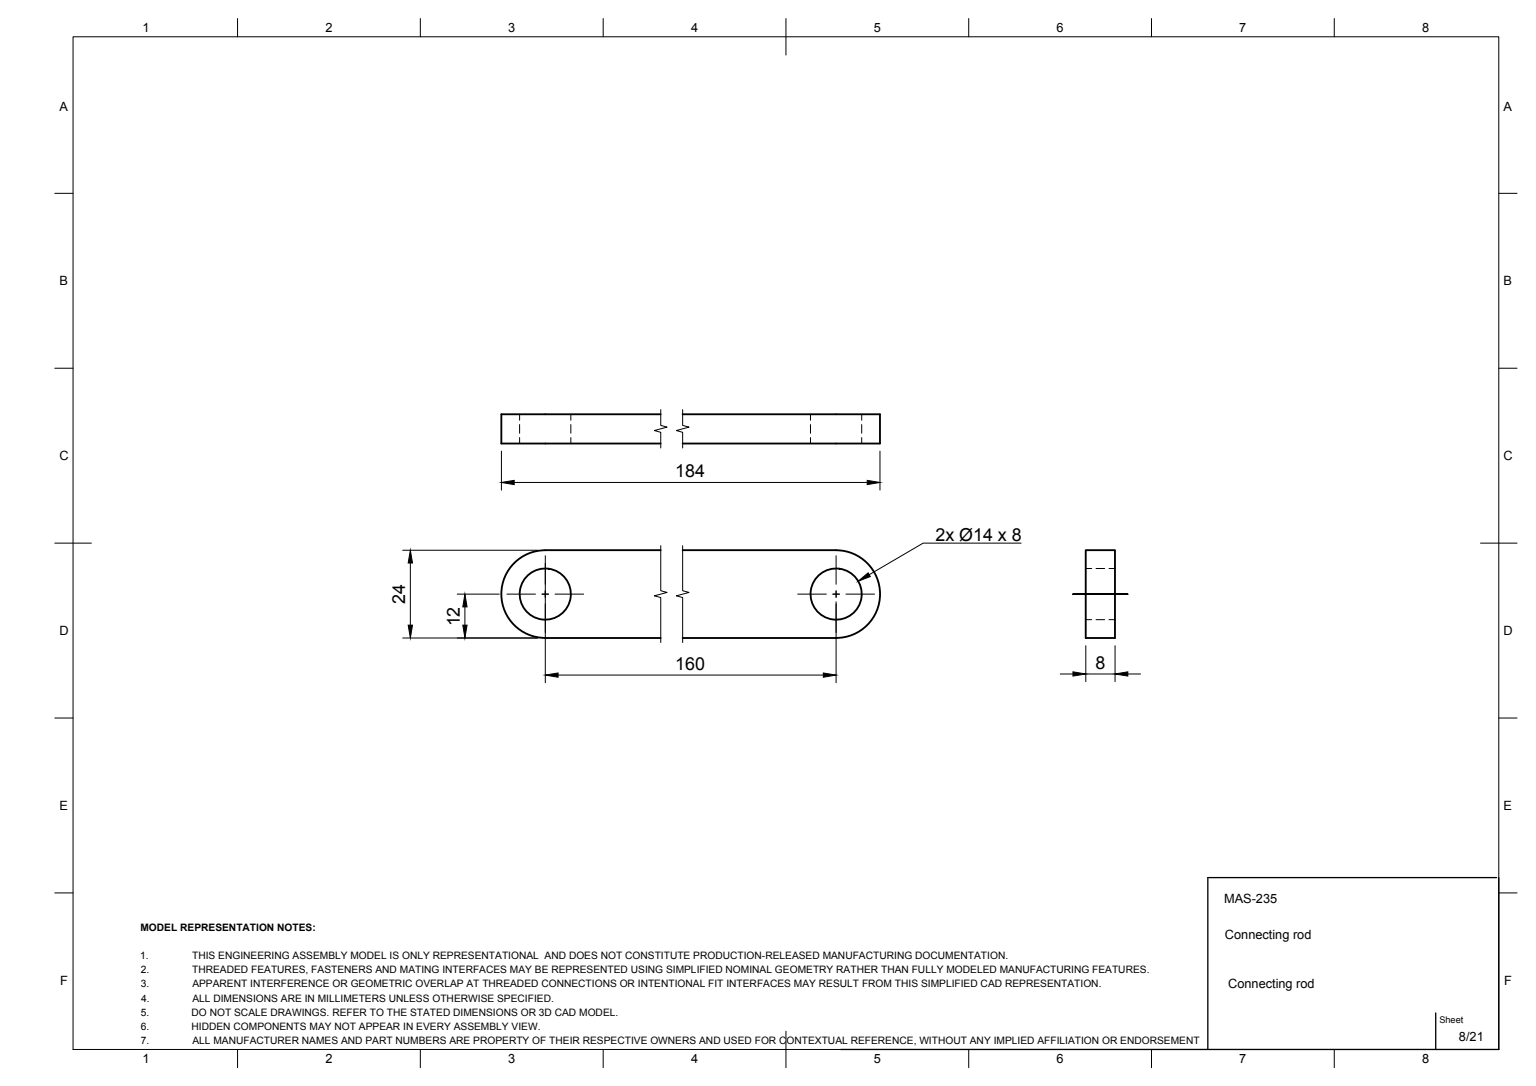
ISO-10303-21;
HEADER;
/* Generated by software containing ST-Developer
 * from STEP Tools, Inc. (www.steptools.com) 
 */

FILE_DESCRIPTION(
/* description */ ('Independent Whitworth quick-return mechanism. Crank radius40, ground-
center spacing80, lever180, connecting rod160, output guide X200. Nomi
nal stroke180 and long/short phase ratio2. Retained guide rods, replac
eable bearing sleeves and captured sliding shoe. No load or production
 rating assigned.'),
/* implementation_level */ '2;1');

FILE_NAME(
/* name */ 'Connecting rod.step',
/* time_stamp */ '2026-11-09T18:22:56-08:00',
/* author */ (''),
/* organization */ (''),
/* preprocessor_version */ 'ST-DEVELOPER v20.2',
/* originating_system */ 'Autodesk Translation Framework v15.17.0.0',
/* authorisation */ '');

FILE_SCHEMA (('AUTOMOTIVE_DESIGN { 1 0 10303 214 3 1 1 }'));
ENDSEC;

DATA;
#10=MECHANICAL_DESIGN_GEOMETRIC_PRESENTATION_REPRESENTATION('',(#224),#4388);
#184=SHAPE_REPRESENTATION_RELATIONSHIP('SRR','None',#4483,#204);
#204=ADVANCED_BREP_SHAPE_REPRESENTATION('',(#244),#4373);
#224=STYLED_ITEM('',(#4591),#244);
#244=MANIFOLD_SOLID_BREP('Body1',#2329);
#277=FACE_BOUND('',#613,.T.);
#278=FACE_BOUND('',#614,.T.);
#279=FACE_BOUND('',#616,.T.);
#280=FACE_BOUND('',#617,.T.);
#339=PLANE('',#2646);
#340=PLANE('',#2650);
#341=PLANE('',#2654);
#342=PLANE('',#2655);
#441=FACE_OUTER_BOUND('',#606,.T.);
#442=FACE_OUTER_BOUND('',#607,.T.);
#443=FACE_OUTER_BOUND('',#608,.T.);
#444=FACE_OUTER_BOUND('',#609,.T.);
#445=FACE_OUTER_BOUND('',#610,.T.);
#446=FACE_OUTER_BOUND('',#611,.T.);
#447=FACE_OUTER_BOUND('',#612,.T.);
#448=FACE_OUTER_BOUND('',#615,.T.);
#606=EDGE_LOOP('',(#1750,#1751,#1752,#1753));
#607=EDGE_LOOP('',(#1754,#1755,#1756,#1757));
#608=EDGE_LOOP('',(#1758,#1759,#1760,#1761));
#609=EDGE_LOOP('',(#1762,#1763,#1764,#1765));
#610=EDGE_LOOP('',(#1766,#1767,#1768,#1769));
#611=EDGE_LOOP('',(#1770,#1771,#1772,#1773));
#612=EDGE_LOOP('',(#1774,#1775,#1776,#1777));
#613=EDGE_LOOP('',(#1778));
#614=EDGE_LOOP('',(#1779));
#615=EDGE_LOOP('',(#1780,#1781,#1782,#1783));
#616=EDGE_LOOP('',(#1784));
#617=EDGE_LOOP('',(#1785));
#805=LINE('',#3877,#944);
#806=LINE('',#3883,#945);
#807=LINE('',#3888,#946);
#808=LINE('',#3890,#947);
#809=LINE('',#3892,#948);
#810=LINE('',#3893,#949);
#811=LINE('',#3899,#950);
#812=LINE('',#3902,#951);
#813=LINE('',#3904,#952);
#814=LINE('',#3905,#953);
#944=VECTOR('',#3097,7.);
#945=VECTOR('',#3104,7.);
#946=VECTOR('',#3109,10.);
#947=VECTOR('',#3110,10.);
#948=VECTOR('',#3111,10.);
#949=VECTOR('',#3112,10.);
#950=VECTOR('',#3119,10.);
#951=VECTOR('',#3122,10.);
#952=VECTOR('',#3123,10.);
#953=VECTOR('',#3124,10.);
#1069=CIRCLE('',#2641,7.);
#1070=CIRCLE('',#2642,7.);
#1071=CIRCLE('',#2644,7.);
#1072=CIRCLE('',#2645,7.);
#1073=CIRCLE('',#2648,12.);
#1074=CIRCLE('',#2649,12.);
#1075=CIRCLE('',#2652,12.);
#1076=CIRCLE('',#2653,12.);
#1211=VERTEX_POINT('',#3874);
#1212=VERTEX_POINT('',#3876);
#1213=VERTEX_POINT('',#3880);
#1214=VERTEX_POINT('',#3882);
#1215=VERTEX_POINT('',#3886);
#1216=VERTEX_POINT('',#3887);
#1217=VERTEX_POINT('',#3889);
#1218=VERTEX_POINT('',#3891);
#1219=VERTEX_POINT('',#3895);
#1220=VERTEX_POINT('',#3897);
#1221=VERTEX_POINT('',#3901);
#1222=VERTEX_POINT('',#3903);
#1411=EDGE_CURVE('',#1211,#1211,#1069,.T.);
#1412=EDGE_CURVE('',#1211,#1212,#805,.T.);
#1413=EDGE_CURVE('',#1212,#1212,#1070,.T.);
#1414=EDGE_CURVE('',#1213,#1213,#1071,.T.);
#1415=EDGE_CURVE('',#1213,#1214,#806,.T.);
#1416=EDGE_CURVE('',#1214,#1214,#1072,.T.);
#1417=EDGE_CURVE('',#1215,#1216,#807,.T.);
#1418=EDGE_CURVE('',#1216,#1217,#808,.T.);
#1419=EDGE_CURVE('',#1218,#1217,#809,.T.);
#1420=EDGE_CURVE('',#1215,#1218,#810,.T.);
#1421=EDGE_CURVE('',#1219,#1215,#1073,.T.);
#1422=EDGE_CURVE('',#1220,#1218,#1074,.T.);
#1423=EDGE_CURVE('',#1219,#1220,#811,.T.);
#1424=EDGE_CURVE('',#1221,#1219,#812,.T.);
#1425=EDGE_CURVE('',#1222,#1220,#813,.T.);
#1426=EDGE_CURVE('',#1221,#1222,#814,.T.);
#1427=EDGE_CURVE('',#1216,#1221,#1075,.T.);
#1428=EDGE_CURVE('',#1217,#1222,#1076,.T.);
#1750=ORIENTED_EDGE('',*,*,#1411,.F.);
#1751=ORIENTED_EDGE('',*,*,#1412,.T.);
#1752=ORIENTED_EDGE('',*,*,#1413,.F.);
#1753=ORIENTED_EDGE('',*,*,#1412,.F.);
#1754=ORIENTED_EDGE('',*,*,#1414,.F.);
#1755=ORIENTED_EDGE('',*,*,#1415,.T.);
#1756=ORIENTED_EDGE('',*,*,#1416,.F.);
#1757=ORIENTED_EDGE('',*,*,#1415,.F.);
#1758=ORIENTED_EDGE('',*,*,#1417,.T.);
#1759=ORIENTED_EDGE('',*,*,#1418,.T.);
#1760=ORIENTED_EDGE('',*,*,#1419,.F.);
#1761=ORIENTED_EDGE('',*,*,#1420,.F.);
#1762=ORIENTED_EDGE('',*,*,#1421,.T.);
#1763=ORIENTED_EDGE('',*,*,#1420,.T.);
#1764=ORIENTED_EDGE('',*,*,#1422,.F.);
#1765=ORIENTED_EDGE('',*,*,#1423,.F.);
#1766=ORIENTED_EDGE('',*,*,#1424,.T.);
#1767=ORIENTED_EDGE('',*,*,#1423,.T.);
#1768=ORIENTED_EDGE('',*,*,#1425,.F.);
#1769=ORIENTED_EDGE('',*,*,#1426,.F.);
#1770=ORIENTED_EDGE('',*,*,#1427,.T.);
#1771=ORIENTED_EDGE('',*,*,#1426,.T.);
#1772=ORIENTED_EDGE('',*,*,#1428,.F.);
#1773=ORIENTED_EDGE('',*,*,#1418,.F.);
#1774=ORIENTED_EDGE('',*,*,#1428,.T.);
#1775=ORIENTED_EDGE('',*,*,#1425,.T.);
#1776=ORIENTED_EDGE('',*,*,#1422,.T.);
#1777=ORIENTED_EDGE('',*,*,#1419,.T.);
#1778=ORIENTED_EDGE('',*,*,#1411,.T.);
#1779=ORIENTED_EDGE('',*,*,#1414,.T.);
#1780=ORIENTED_EDGE('',*,*,#1427,.F.);
#1781=ORIENTED_EDGE('',*,*,#1417,.F.);
#1782=ORIENTED_EDGE('',*,*,#1421,.F.);
#1783=ORIENTED_EDGE('',*,*,#1424,.F.);
#1784=ORIENTED_EDGE('',*,*,#1413,.T.);
#1785=ORIENTED_EDGE('',*,*,#1416,.T.);
#2132=CYLINDRICAL_SURFACE('',#2640,7.);
#2133=CYLINDRICAL_SURFACE('',#2643,7.);
#2134=CYLINDRICAL_SURFACE('',#2647,12.);
#2135=CYLINDRICAL_SURFACE('',#2651,12.);
#2213=ADVANCED_FACE('',(#441),#2132,.F.);
#2214=ADVANCED_FACE('',(#442),#2133,.F.);
#2215=ADVANCED_FACE('',(#443),#339,.T.);
#2216=ADVANCED_FACE('',(#444),#2134,.T.);
#2217=ADVANCED_FACE('',(#445),#340,.T.);
#2218=ADVANCED_FACE('',(#446),#2135,.T.);
#2219=ADVANCED_FACE('',(#447,#277,#278),#341,.T.);
#2220=ADVANCED_FACE('',(#448,#279,#280),#342,.F.);
#2329=CLOSED_SHELL('',(#2213,#2214,#2215,#2216,#2217,#2218,#2219,#2220));
#2639=AXIS2_PLACEMENT_3D('',#3872,#3091,#3092);
#2640=AXIS2_PLACEMENT_3D('',#3873,#3093,#3094);
#2641=AXIS2_PLACEMENT_3D('',#3875,#3095,#3096);
#2642=AXIS2_PLACEMENT_3D('',#3878,#3098,#3099);
#2643=AXIS2_PLACEMENT_3D('',#3879,#3100,#3101);
#2644=AXIS2_PLACEMENT_3D('',#3881,#3102,#3103);
#2645=AXIS2_PLACEMENT_3D('',#3884,#3105,#3106);
#2646=AXIS2_PLACEMENT_3D('',#3885,#3107,#3108);
#2647=AXIS2_PLACEMENT_3D('',#3894,#3113,#3114);
#2648=AXIS2_PLACEMENT_3D('',#3896,#3115,#3116);
#2649=AXIS2_PLACEMENT_3D('',#3898,#3117,#3118);
#2650=AXIS2_PLACEMENT_3D('',#3900,#3120,#3121);
#2651=AXIS2_PLACEMENT_3D('',#3906,#3125,#3126);
#2652=AXIS2_PLACEMENT_3D('',#3907,#3127,#3128);
#2653=AXIS2_PLACEMENT_3D('',#3908,#3129,#3130);
#2654=AXIS2_PLACEMENT_3D('',#3909,#3131,#3132);
#2655=AXIS2_PLACEMENT_3D('',#3910,#3133,#3134);
#3091=DIRECTION('axis',(0.,0.,1.));
#3092=DIRECTION('refdir',(1.,0.,0.));
#3093=DIRECTION('center_axis',(0.,0.,-1.));
#3094=DIRECTION('ref_axis',(1.,0.,0.));
#3095=DIRECTION('center_axis',(0.,0.,-1.));
#3096=DIRECTION('ref_axis',(1.,0.,0.));
#3097=DIRECTION('',(0.,0.,-1.));
#3098=DIRECTION('center_axis',(0.,0.,1.));
#3099=DIRECTION('ref_axis',(1.,0.,0.));
#3100=DIRECTION('center_axis',(0.,0.,-1.));
#3101=DIRECTION('ref_axis',(1.,0.,0.));
#3102=DIRECTION('center_axis',(0.,0.,-1.));
#3103=DIRECTION('ref_axis',(1.,0.,0.));
#3104=DIRECTION('',(0.,0.,-1.));
#3105=DIRECTION('center_axis',(0.,0.,1.));
#3106=DIRECTION('ref_axis',(1.,0.,0.));
#3107=DIRECTION('center_axis',(0.,1.,0.));
#3108=DIRECTION('ref_axis',(-1.,0.,0.));
#3109=DIRECTION('',(-1.,0.,0.));
#3110=DIRECTION('',(0.,0.,1.));
#3111=DIRECTION('',(-1.,0.,0.));
#3112=DIRECTION('',(0.,0.,1.));
#3113=DIRECTION('center_axis',(0.,0.,1.));
#3114=DIRECTION('ref_axis',(0.,-1.,0.));
#3115=DIRECTION('center_axis',(0.,0.,1.));
#3116=DIRECTION('ref_axis',(0.,-1.,0.));
#3117=DIRECTION('center_axis',(0.,0.,1.));
#3118=DIRECTION('ref_axis',(0.,-1.,0.));
#3119=DIRECTION('',(0.,0.,1.));
#3120=DIRECTION('center_axis',(0.,-1.,0.));
#3121=DIRECTION('ref_axis',(1.,0.,0.));
#3122=DIRECTION('',(1.,0.,0.));
#3123=DIRECTION('',(1.,0.,0.));
#3124=DIRECTION('',(0.,0.,1.));
#3125=DIRECTION('center_axis',(0.,0.,1.));
#3126=DIRECTION('ref_axis',(0.,1.,0.));
#3127=DIRECTION('center_axis',(0.,0.,1.));
#3128=DIRECTION('ref_axis',(0.,1.,0.));
#3129=DIRECTION('center_axis',(0.,0.,1.));
#3130=DIRECTION('ref_axis',(0.,1.,0.));
#3131=DIRECTION('center_axis',(0.,0.,1.));
#3132=DIRECTION('ref_axis',(1.,0.,0.));
#3133=DIRECTION('center_axis',(0.,0.,1.));
#3134=DIRECTION('ref_axis',(1.,0.,0.));
#3872=CARTESIAN_POINT('',(0.,0.,0.));
#3873=CARTESIAN_POINT('Origin',(0.,0.,4.));
#3874=CARTESIAN_POINT('',(-7.,8.57252759403147E-16,8.));
#3875=CARTESIAN_POINT('Origin',(0.,0.,8.));
#3876=CARTESIAN_POINT('',(-7.,8.57252759403147E-16,0.));
#3877=CARTESIAN_POINT('',(-7.,8.57252759403147E-16,4.));
#3878=CARTESIAN_POINT('Origin',(0.,0.,0.));
#3879=CARTESIAN_POINT('Origin',(160.,0.,4.));
#3880=CARTESIAN_POINT('',(153.,8.57252759403147E-16,8.));
#3881=CARTESIAN_POINT('Origin',(160.,0.,8.));
#3882=CARTESIAN_POINT('',(153.,8.57252759403147E-16,0.));
#3883=CARTESIAN_POINT('',(153.,8.57252759403147E-16,4.));
#3884=CARTESIAN_POINT('Origin',(160.,0.,0.));
#3885=CARTESIAN_POINT('Origin',(160.,12.,0.));
#3886=CARTESIAN_POINT('',(160.,12.,0.));
#3887=CARTESIAN_POINT('',(0.,12.,0.));
#3888=CARTESIAN_POINT('',(160.,12.,0.));
#3889=CARTESIAN_POINT('',(0.,12.,8.));
#3890=CARTESIAN_POINT('',(0.,12.,0.));
#3891=CARTESIAN_POINT('',(160.,12.,8.));
#3892=CARTESIAN_POINT('',(160.,12.,8.));
#3893=CARTESIAN_POINT('',(160.,12.,0.));
#3894=CARTESIAN_POINT('Origin',(160.,-1.11022302462516E-15,0.));
#3895=CARTESIAN_POINT('',(160.,-12.,0.));
#3896=CARTESIAN_POINT('Origin',(160.,-1.11022302462516E-15,0.));
#3897=CARTESIAN_POINT('',(160.,-12.,8.));
#3898=CARTESIAN_POINT('Origin',(160.,-1.11022302462516E-15,8.));
#3899=CARTESIAN_POINT('',(160.,-12.,0.));
#3900=CARTESIAN_POINT('Origin',(0.,-12.,0.));
#3901=CARTESIAN_POINT('',(-1.46957615897682E-15,-12.,0.));
#3902=CARTESIAN_POINT('',(0.,-12.,0.));
#3903=CARTESIAN_POINT('',(-1.46957615897682E-15,-12.,8.));
#3904=CARTESIAN_POINT('',(0.,-12.,8.));
#3905=CARTESIAN_POINT('',(-1.46957615897682E-15,-12.,0.));
#3906=CARTESIAN_POINT('Origin',(0.,0.,0.));
#3907=CARTESIAN_POINT('Origin',(0.,0.,0.));
#3908=CARTESIAN_POINT('Origin',(0.,0.,8.));
#3909=CARTESIAN_POINT('Origin',(80.,0.,8.));
#3910=CARTESIAN_POINT('Origin',(80.,0.,0.));
#4351=UNCERTAINTY_MEASURE_WITH_UNIT(LENGTH_MEASURE(0.01),#4389,
'DISTANCE_ACCURACY_VALUE',
'Maximum model space distance between geometric entities at asserted c
onnectivities');
#4366=UNCERTAINTY_MEASURE_WITH_UNIT(LENGTH_MEASURE(0.01),#4389,
'DISTANCE_ACCURACY_VALUE',
'Maximum model space distance between geometric entities at asserted c
onnectivities');
#4373=(
GEOMETRIC_REPRESENTATION_CONTEXT(3)
GLOBAL_UNCERTAINTY_ASSIGNED_CONTEXT((#4351))
GLOBAL_UNIT_ASSIGNED_CONTEXT((#4389,#4391,#4392))
REPRESENTATION_CONTEXT('','3D')
);
#4388=(
GEOMETRIC_REPRESENTATION_CONTEXT(3)
GLOBAL_UNCERTAINTY_ASSIGNED_CONTEXT((#4366))
GLOBAL_UNIT_ASSIGNED_CONTEXT((#4389,#4391,#4392))
REPRESENTATION_CONTEXT('','3D')
);
#4389=(
LENGTH_UNIT()
NAMED_UNIT(*)
SI_UNIT(.MILLI.,.METRE.)
);
#4391=(
NAMED_UNIT(*)
PLANE_ANGLE_UNIT()
SI_UNIT($,.RADIAN.)
);
#4392=(
NAMED_UNIT(*)
SI_UNIT($,.STERADIAN.)
SOLID_ANGLE_UNIT()
);
#4399=SHAPE_DEFINITION_REPRESENTATION(#4420,#4483);
#4420=PRODUCT_DEFINITION_SHAPE('',$,#4505);
#4483=SHAPE_REPRESENTATION('',(#2639),#4373);
#4498=PRODUCT_DEFINITION_CONTEXT('part definition',#4563,'design');
#4505=PRODUCT_DEFINITION('Connecting rod','Connecting rod',#4526,#4498);
#4526=PRODUCT_DEFINITION_FORMATION('',$,#4571);
#4563=APPLICATION_CONTEXT(
'Core Data for Automotive Mechanical Design Process');
#4564=PRODUCT_CONTEXT('part definition',#4563,'mechanical');
#4571=PRODUCT('Connecting rod','Connecting rod','Connecting rod',(#4564));
#4591=PRESENTATION_STYLE_ASSIGNMENT((#4605));
#4605=SURFACE_STYLE_USAGE(.BOTH.,#4619);
#4619=SURFACE_SIDE_STYLE('',(#4633));
#4633=SURFACE_STYLE_FILL_AREA(#4647);
#4647=FILL_AREA_STYLE('Connecting rod finish',(#4661));
#4661=FILL_AREA_STYLE_COLOUR('Connecting rod finish',#4675);
#4675=COLOUR_RGB('Connecting rod finish',0.662745098039216,0.831372549019608,
0.949019607843137);
ENDSEC;
END-ISO-10303-21;
